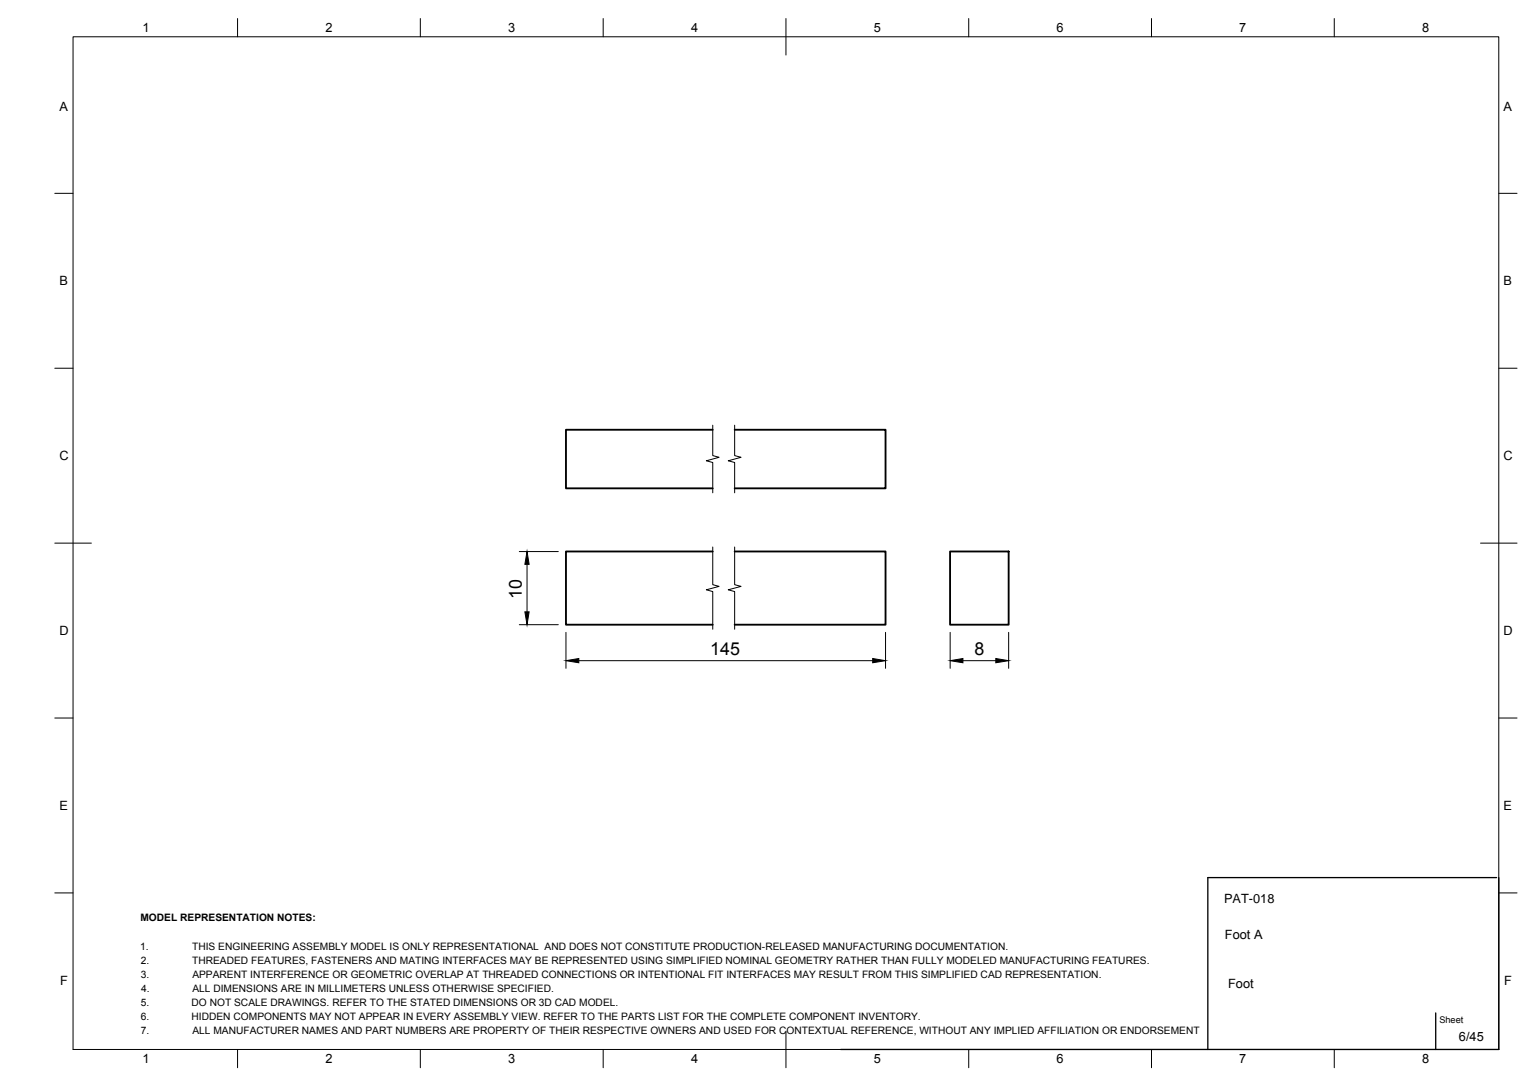
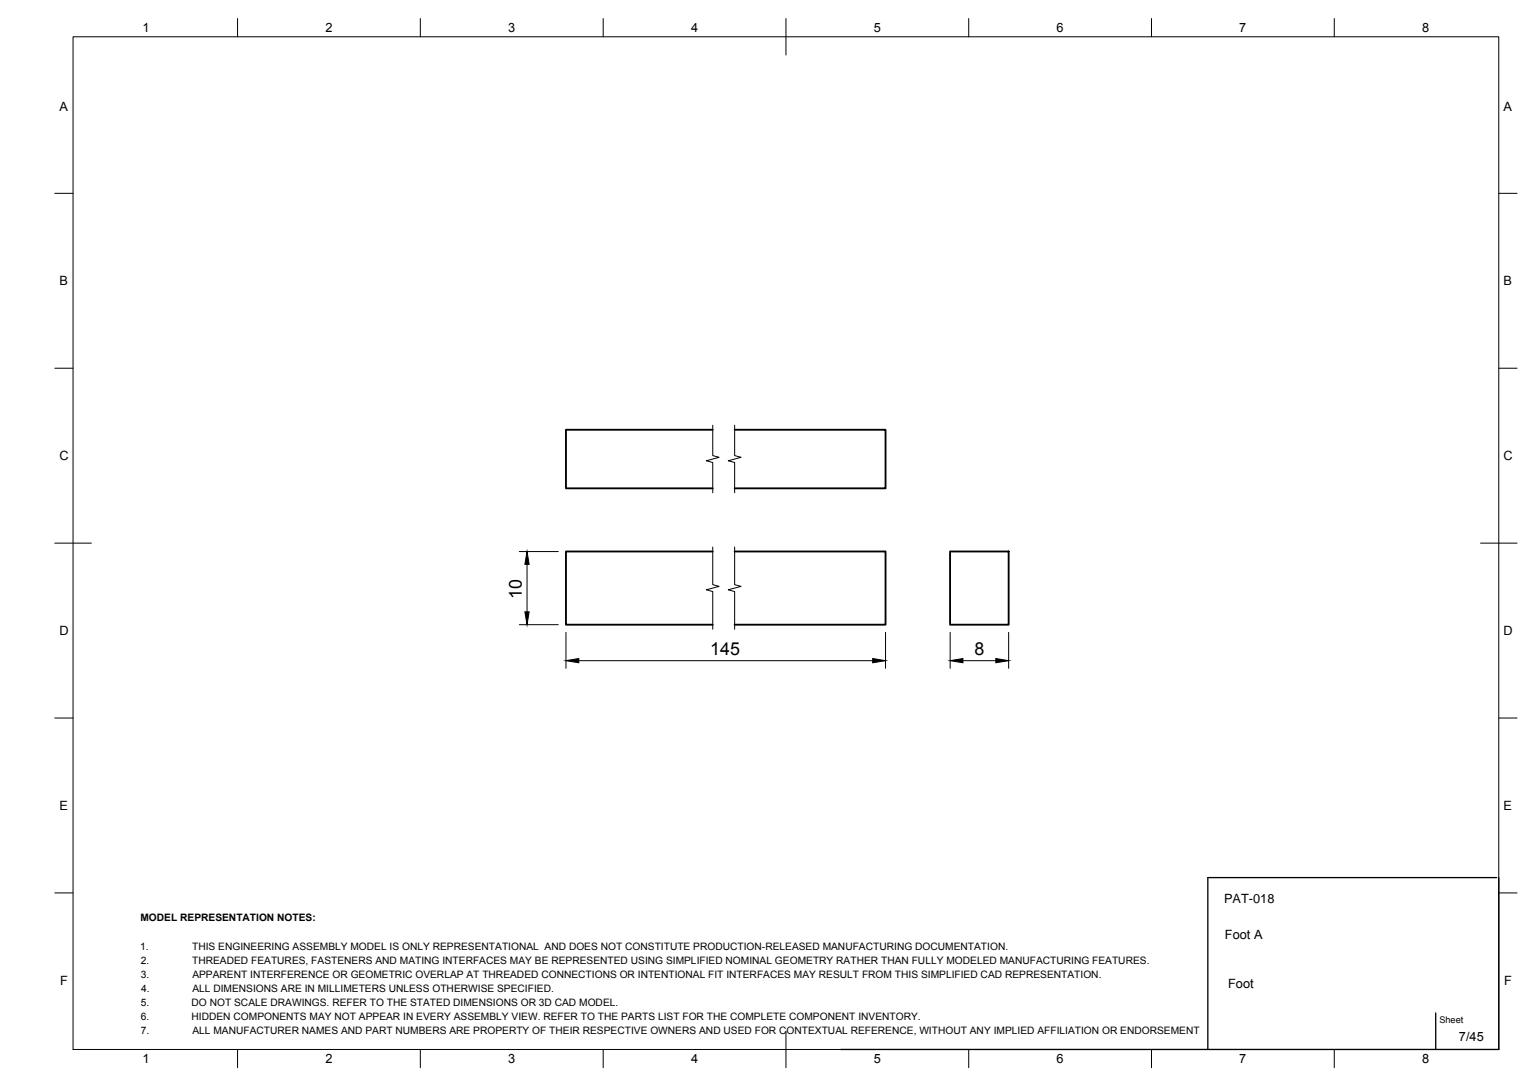
ISO-10303-21;
HEADER;
/* Generated by software containing ST-Developer
 * from STEP Tools, Inc. (www.steptools.com) 
 */

FILE_DESCRIPTION(
/* description */ ('Cam-driven reciprocating slide'),
/* implementation_level */ '2;1');

FILE_NAME(
/* name */ 'Foot.step',
/* time_stamp */ '2026-10-28T03:25:20-07:00',
/* author */ (''),
/* organization */ (''),
/* preprocessor_version */ 'ST-DEVELOPER v20.2',
/* originating_system */ 'Autodesk Translation Framework v15.17.0.0',
/* authorisation */ '');

FILE_SCHEMA (('AUTOMOTIVE_DESIGN { 1 0 10303 214 3 1 1 }'));
ENDSEC;

DATA;
#10=MECHANICAL_DESIGN_GEOMETRIC_PRESENTATION_REPRESENTATION('',(#423),#13277);
#349=SHAPE_REPRESENTATION_RELATIONSHIP('SRR','None',#13442,#386);
#386=ADVANCED_BREP_SHAPE_REPRESENTATION('',(#467),#13237);
#423=STYLED_ITEM('',(#13734),#467);
#467=MANIFOLD_SOLID_BREP('Body1',#6399);
#692=PLANE('',#6886);
#693=PLANE('',#6887);
#694=PLANE('',#6888);
#695=PLANE('',#6889);
#696=PLANE('',#6890);
#697=PLANE('',#6891);
#918=FACE_OUTER_BOUND('',#1310,.T.);
#919=FACE_OUTER_BOUND('',#1311,.T.);
#920=FACE_OUTER_BOUND('',#1312,.T.);
#921=FACE_OUTER_BOUND('',#1313,.T.);
#922=FACE_OUTER_BOUND('',#1314,.T.);
#923=FACE_OUTER_BOUND('',#1315,.T.);
#1310=EDGE_LOOP('',(#4420,#4421,#4422,#4423));
#1311=EDGE_LOOP('',(#4424,#4425,#4426,#4427));
#1312=EDGE_LOOP('',(#4428,#4429,#4430,#4431));
#1313=EDGE_LOOP('',(#4432,#4433,#4434,#4435));
#1314=EDGE_LOOP('',(#4436,#4437,#4438,#4439));
#1315=EDGE_LOOP('',(#4440,#4441,#4442,#4443));
#1863=LINE('',#9834,#2302);
#1864=LINE('',#9836,#2303);
#1865=LINE('',#9838,#2304);
#1866=LINE('',#9839,#2305);
#1867=LINE('',#9842,#2306);
#1868=LINE('',#9844,#2307);
#1869=LINE('',#9845,#2308);
#1870=LINE('',#9848,#2309);
#1871=LINE('',#9850,#2310);
#1872=LINE('',#9851,#2311);
#1873=LINE('',#9853,#2312);
#1874=LINE('',#9854,#2313);
#2302=VECTOR('',#7767,1.);
#2303=VECTOR('',#7768,1.);
#2304=VECTOR('',#7769,1.);
#2305=VECTOR('',#7770,1.);
#2306=VECTOR('',#7773,1.);
#2307=VECTOR('',#7774,1.);
#2308=VECTOR('',#7775,1.);
#2309=VECTOR('',#7778,1.);
#2310=VECTOR('',#7779,1.);
#2311=VECTOR('',#7780,1.);
#2312=VECTOR('',#7783,1.);
#2313=VECTOR('',#7784,1.);
#3063=VERTEX_POINT('',#9832);
#3064=VERTEX_POINT('',#9833);
#3065=VERTEX_POINT('',#9835);
#3066=VERTEX_POINT('',#9837);
#3067=VERTEX_POINT('',#9841);
#3068=VERTEX_POINT('',#9843);
#3069=VERTEX_POINT('',#9847);
#3070=VERTEX_POINT('',#9849);
#3600=EDGE_CURVE('',#3063,#3064,#1863,.T.);
#3601=EDGE_CURVE('',#3064,#3065,#1864,.T.);
#3602=EDGE_CURVE('',#3066,#3065,#1865,.T.);
#3603=EDGE_CURVE('',#3063,#3066,#1866,.T.);
#3604=EDGE_CURVE('',#3067,#3063,#1867,.T.);
#3605=EDGE_CURVE('',#3068,#3066,#1868,.T.);
#3606=EDGE_CURVE('',#3067,#3068,#1869,.T.);
#3607=EDGE_CURVE('',#3069,#3067,#1870,.T.);
#3608=EDGE_CURVE('',#3070,#3068,#1871,.T.);
#3609=EDGE_CURVE('',#3069,#3070,#1872,.T.);
#3610=EDGE_CURVE('',#3064,#3069,#1873,.T.);
#3611=EDGE_CURVE('',#3065,#3070,#1874,.T.);
#4420=ORIENTED_EDGE('',*,*,#3600,.T.);
#4421=ORIENTED_EDGE('',*,*,#3601,.T.);
#4422=ORIENTED_EDGE('',*,*,#3602,.F.);
#4423=ORIENTED_EDGE('',*,*,#3603,.F.);
#4424=ORIENTED_EDGE('',*,*,#3604,.T.);
#4425=ORIENTED_EDGE('',*,*,#3603,.T.);
#4426=ORIENTED_EDGE('',*,*,#3605,.F.);
#4427=ORIENTED_EDGE('',*,*,#3606,.F.);
#4428=ORIENTED_EDGE('',*,*,#3607,.T.);
#4429=ORIENTED_EDGE('',*,*,#3606,.T.);
#4430=ORIENTED_EDGE('',*,*,#3608,.F.);
#4431=ORIENTED_EDGE('',*,*,#3609,.F.);
#4432=ORIENTED_EDGE('',*,*,#3610,.T.);
#4433=ORIENTED_EDGE('',*,*,#3609,.T.);
#4434=ORIENTED_EDGE('',*,*,#3611,.F.);
#4435=ORIENTED_EDGE('',*,*,#3601,.F.);
#4436=ORIENTED_EDGE('',*,*,#3611,.T.);
#4437=ORIENTED_EDGE('',*,*,#3608,.T.);
#4438=ORIENTED_EDGE('',*,*,#3605,.T.);
#4439=ORIENTED_EDGE('',*,*,#3602,.T.);
#4440=ORIENTED_EDGE('',*,*,#3610,.F.);
#4441=ORIENTED_EDGE('',*,*,#3600,.F.);
#4442=ORIENTED_EDGE('',*,*,#3604,.F.);
#4443=ORIENTED_EDGE('',*,*,#3607,.F.);
#6036=ADVANCED_FACE('',(#918),#692,.T.);
#6037=ADVANCED_FACE('',(#919),#693,.T.);
#6038=ADVANCED_FACE('',(#920),#694,.T.);
#6039=ADVANCED_FACE('',(#921),#695,.T.);
#6040=ADVANCED_FACE('',(#922),#696,.T.);
#6041=ADVANCED_FACE('',(#923),#697,.F.);
#6399=CLOSED_SHELL('',(#6036,#6037,#6038,#6039,#6040,#6041));
#6885=AXIS2_PLACEMENT_3D('',#9830,#7763,#7764);
#6886=AXIS2_PLACEMENT_3D('',#9831,#7765,#7766);
#6887=AXIS2_PLACEMENT_3D('',#9840,#7771,#7772);
#6888=AXIS2_PLACEMENT_3D('',#9846,#7776,#7777);
#6889=AXIS2_PLACEMENT_3D('',#9852,#7781,#7782);
#6890=AXIS2_PLACEMENT_3D('',#9855,#7785,#7786);
#6891=AXIS2_PLACEMENT_3D('',#9856,#7787,#7788);
#7763=DIRECTION('axis',(0.,0.,1.));
#7764=DIRECTION('refdir',(1.,0.,0.));
#7765=DIRECTION('center_axis',(0.,1.,0.));
#7766=DIRECTION('ref_axis',(-1.,0.,0.));
#7767=DIRECTION('',(-1.,0.,0.));
#7768=DIRECTION('',(0.,0.,1.));
#7769=DIRECTION('',(-1.,0.,0.));
#7770=DIRECTION('',(0.,0.,1.));
#7771=DIRECTION('center_axis',(1.,0.,0.));
#7772=DIRECTION('ref_axis',(0.,1.,0.));
#7773=DIRECTION('',(0.,1.,0.));
#7774=DIRECTION('',(0.,1.,0.));
#7775=DIRECTION('',(0.,0.,1.));
#7776=DIRECTION('center_axis',(0.,-1.,0.));
#7777=DIRECTION('ref_axis',(1.,0.,0.));
#7778=DIRECTION('',(1.,0.,0.));
#7779=DIRECTION('',(1.,0.,0.));
#7780=DIRECTION('',(0.,0.,1.));
#7781=DIRECTION('center_axis',(-1.,0.,0.));
#7782=DIRECTION('ref_axis',(0.,-1.,0.));
#7783=DIRECTION('',(0.,-1.,0.));
#7784=DIRECTION('',(0.,-1.,0.));
#7785=DIRECTION('center_axis',(0.,0.,1.));
#7786=DIRECTION('ref_axis',(1.,0.,0.));
#7787=DIRECTION('center_axis',(0.,0.,1.));
#7788=DIRECTION('ref_axis',(1.,0.,0.));
#9830=CARTESIAN_POINT('',(0.,0.,0.));
#9831=CARTESIAN_POINT('Origin',(-5.,9.,-0.8));
#9832=CARTESIAN_POINT('',(-5.,9.,-0.8));
#9833=CARTESIAN_POINT('',(-6.,9.,-0.8));
#9834=CARTESIAN_POINT('',(-5.,9.,-0.8));
#9835=CARTESIAN_POINT('',(-6.,9.,0.));
#9836=CARTESIAN_POINT('',(-6.,9.,-0.8));
#9837=CARTESIAN_POINT('',(-5.,9.,0.));
#9838=CARTESIAN_POINT('',(-5.,9.,0.));
#9839=CARTESIAN_POINT('',(-5.,9.,-0.8));
#9840=CARTESIAN_POINT('Origin',(-5.,-5.5,-0.8));
#9841=CARTESIAN_POINT('',(-5.,-5.5,-0.8));
#9842=CARTESIAN_POINT('',(-5.,-5.5,-0.8));
#9843=CARTESIAN_POINT('',(-5.,-5.5,0.));
#9844=CARTESIAN_POINT('',(-5.,-5.5,0.));
#9845=CARTESIAN_POINT('',(-5.,-5.5,-0.8));
#9846=CARTESIAN_POINT('Origin',(-6.,-5.5,-0.8));
#9847=CARTESIAN_POINT('',(-6.,-5.5,-0.8));
#9848=CARTESIAN_POINT('',(-6.,-5.5,-0.8));
#9849=CARTESIAN_POINT('',(-6.,-5.5,0.));
#9850=CARTESIAN_POINT('',(-6.,-5.5,0.));
#9851=CARTESIAN_POINT('',(-6.,-5.5,-0.8));
#9852=CARTESIAN_POINT('Origin',(-6.,9.,-0.8));
#9853=CARTESIAN_POINT('',(-6.,9.,-0.8));
#9854=CARTESIAN_POINT('',(-6.,9.,0.));
#9855=CARTESIAN_POINT('Origin',(-5.5,1.75,0.));
#9856=CARTESIAN_POINT('Origin',(-5.5,1.75,-0.8));
#13193=UNCERTAINTY_MEASURE_WITH_UNIT(LENGTH_MEASURE(0.001),#13278,
'DISTANCE_ACCURACY_VALUE',
'Maximum model space distance between geometric entities at asserted c
onnectivities');
#13233=UNCERTAINTY_MEASURE_WITH_UNIT(LENGTH_MEASURE(0.001),#13278,
'DISTANCE_ACCURACY_VALUE',
'Maximum model space distance between geometric entities at asserted c
onnectivities');
#13237=(
GEOMETRIC_REPRESENTATION_CONTEXT(3)
GLOBAL_UNCERTAINTY_ASSIGNED_CONTEXT((#13193))
GLOBAL_UNIT_ASSIGNED_CONTEXT((#13278,#13280,#13281))
REPRESENTATION_CONTEXT('','3D')
);
#13277=(
GEOMETRIC_REPRESENTATION_CONTEXT(3)
GLOBAL_UNCERTAINTY_ASSIGNED_CONTEXT((#13233))
GLOBAL_UNIT_ASSIGNED_CONTEXT((#13278,#13280,#13281))
REPRESENTATION_CONTEXT('','3D')
);
#13278=(
LENGTH_UNIT()
NAMED_UNIT(*)
SI_UNIT(.CENTI.,.METRE.)
);
#13280=(
NAMED_UNIT(*)
PLANE_ANGLE_UNIT()
SI_UNIT($,.RADIAN.)
);
#13281=(
NAMED_UNIT(*)
SI_UNIT($,.STERADIAN.)
SOLID_ANGLE_UNIT()
);
#13285=SHAPE_DEFINITION_REPRESENTATION(#13328,#13442);
#13328=PRODUCT_DEFINITION_SHAPE('',$,#13486);
#13442=SHAPE_REPRESENTATION('',(#6885),#13237);
#13482=PRODUCT_DEFINITION_CONTEXT('part definition',#13613,'design');
#13486=PRODUCT_DEFINITION('Foot','Foot',#13529,#13482);
#13529=PRODUCT_DEFINITION_FORMATION('',$,#13618);
#13613=APPLICATION_CONTEXT(
'Core Data for Automotive Mechanical Design Process');
#13614=PRODUCT_CONTEXT('part definition',#13613,'mechanical');
#13618=PRODUCT('Foot','Foot','Foot',(#13614));
#13728=COLOUR_RGB('Off White',0.89,0.88,0.83);
#13729=FILL_AREA_STYLE_COLOUR('',#13728);
#13730=FILL_AREA_STYLE('',(#13729));
#13731=SURFACE_STYLE_FILL_AREA(#13730);
#13732=SURFACE_SIDE_STYLE('',(#13731));
#13733=SURFACE_STYLE_USAGE(.BOTH.,#13732);
#13734=PRESENTATION_STYLE_ASSIGNMENT((#13733));
ENDSEC;
END-ISO-10303-21;
